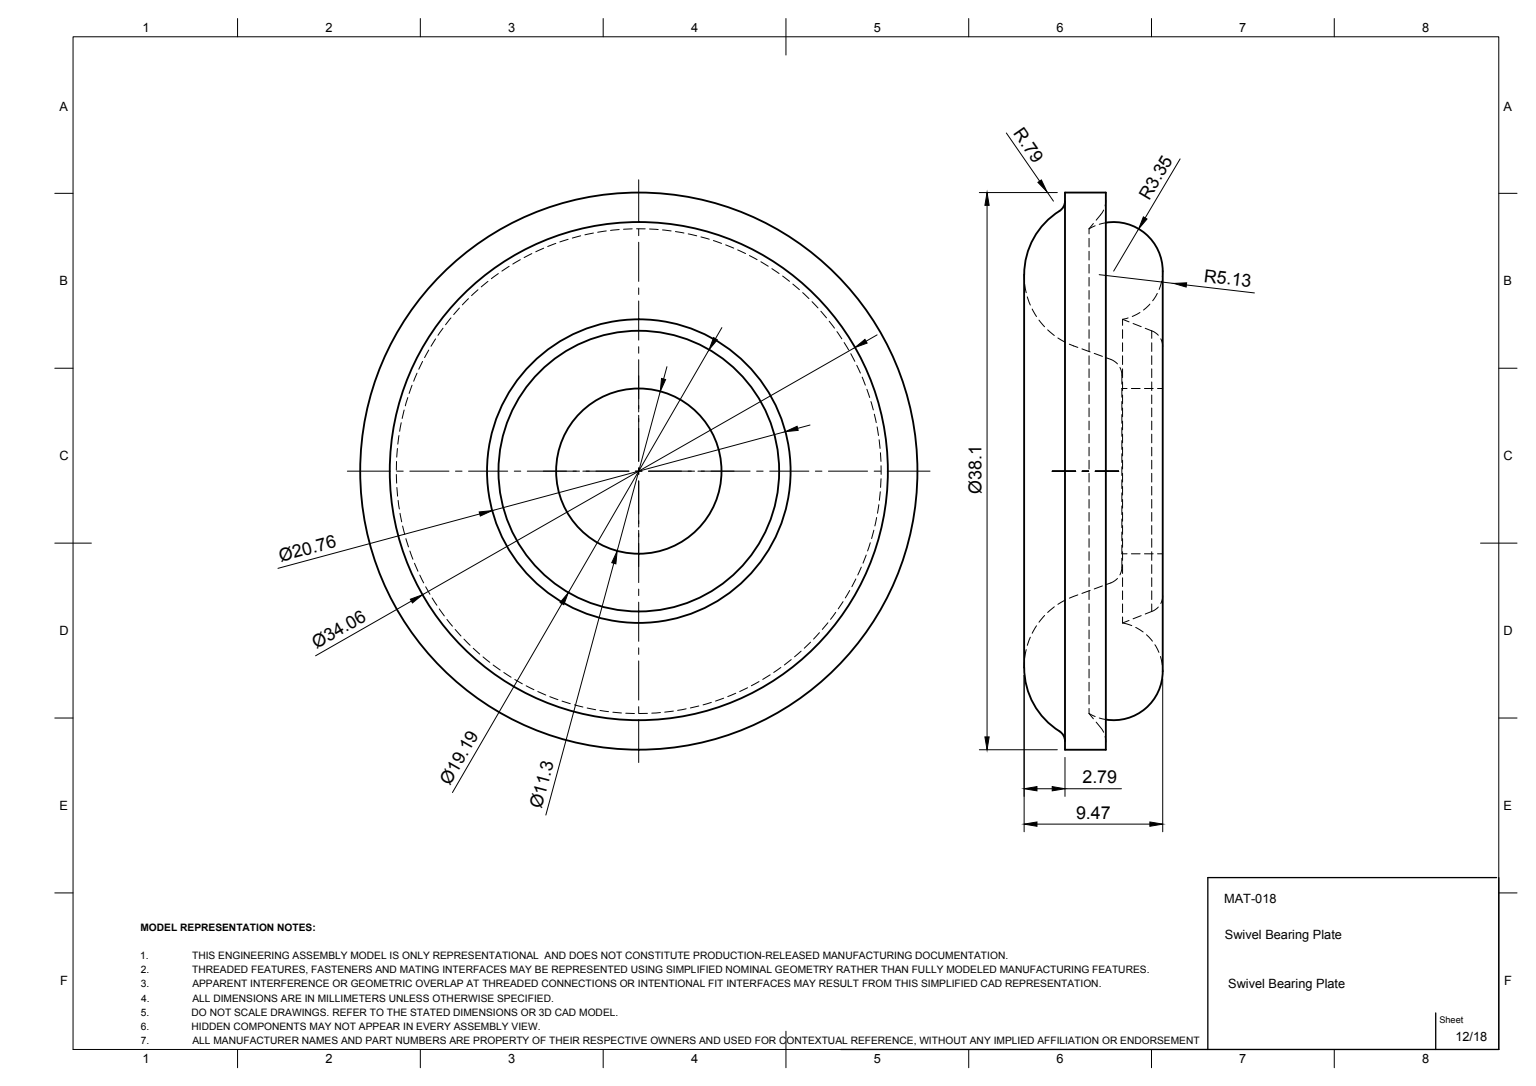
ISO-10303-21;
HEADER;
/* Generated by software containing ST-Developer
 * from STEP Tools, Inc. (www.steptools.com) 
 */

FILE_DESCRIPTION(
/* description */ ('STEP AP214'),
/* implementation_level */ '2;1');

FILE_NAME(
/* name */ 'Swivel Bearing Plate.step',
/* time_stamp */ '2026-11-14T06:16:09-08:00',
/* author */ (''),
/* organization */ (''),
/* preprocessor_version */ 'ST-DEVELOPER v20.2',
/* originating_system */ 'Autodesk Translation Framework v15.17.0.0',
/* authorisation */ '');

FILE_SCHEMA (('AUTOMOTIVE_DESIGN { 1 0 10303 214 3 1 1 }'));
ENDSEC;

DATA;
#10=MECHANICAL_DESIGN_GEOMETRIC_PRESENTATION_REPRESENTATION('',(#355),#18006);
#126=CONICAL_SURFACE('',#10555,9.59611131114252,0.375229267578829);
#127=CONICAL_SURFACE('',#10558,15.3208607241417,0.87573749484567);
#128=CONICAL_SURFACE('',#10579,8.56864389726312,0.349065850398865);
#241=TOROIDAL_SURFACE('',#10550,8.52204264558423,1.143);
#242=TOROIDAL_SURFACE('',#10561,18.5282252464232,1.5748);
#243=TOROIDAL_SURFACE('',#10567,18.4629769854638,0.7874);
#244=TOROIDAL_SURFACE('',#10571,13.4366,5.1308);
#245=TOROIDAL_SURFACE('',#10574,13.3900187959915,5.1308);
#246=TOROIDAL_SURFACE('',#10582,6.5656627838263,1.143);
#247=TOROIDAL_SURFACE('',#10585,13.6779,3.3528);
#323=SHAPE_REPRESENTATION_RELATIONSHIP('SRR','None',#18081,#339);
#339=ADVANCED_BREP_SHAPE_REPRESENTATION('',(#371),#17998);
#355=STYLED_ITEM('',(#18172),#371);
#371=MANIFOLD_SOLID_BREP('Body1',#9564);
#471=FACE_BOUND('',#1968,.T.);
#472=FACE_BOUND('',#1970,.T.);
#473=FACE_BOUND('',#1972,.T.);
#474=FACE_BOUND('',#1974,.T.);
#475=FACE_BOUND('',#1976,.T.);
#786=PLANE('',#10587);
#787=PLANE('',#10588);
#788=PLANE('',#10589);
#789=PLANE('',#10590);
#790=PLANE('',#10591);
#1287=FACE_OUTER_BOUND('',#1955,.T.);
#1288=FACE_OUTER_BOUND('',#1956,.T.);
#1289=FACE_OUTER_BOUND('',#1957,.T.);
#1290=FACE_OUTER_BOUND('',#1958,.T.);
#1291=FACE_OUTER_BOUND('',#1959,.T.);
#1292=FACE_OUTER_BOUND('',#1960,.T.);
#1293=FACE_OUTER_BOUND('',#1961,.T.);
#1294=FACE_OUTER_BOUND('',#1962,.T.);
#1295=FACE_OUTER_BOUND('',#1963,.T.);
#1296=FACE_OUTER_BOUND('',#1964,.T.);
#1297=FACE_OUTER_BOUND('',#1965,.T.);
#1298=FACE_OUTER_BOUND('',#1966,.T.);
#1299=FACE_OUTER_BOUND('',#1967,.T.);
#1300=FACE_OUTER_BOUND('',#1969,.T.);
#1301=FACE_OUTER_BOUND('',#1971,.T.);
#1302=FACE_OUTER_BOUND('',#1973,.T.);
#1303=FACE_OUTER_BOUND('',#1975,.T.);
#1955=EDGE_LOOP('',(#8296,#8297,#8298,#8299));
#1956=EDGE_LOOP('',(#8300,#8301,#8302,#8303,#8304));
#1957=EDGE_LOOP('',(#8305,#8306,#8307,#8308,#8309,#8310));
#1958=EDGE_LOOP('',(#8311,#8312,#8313,#8314));
#1959=EDGE_LOOP('',(#8315,#8316,#8317,#8318));
#1960=EDGE_LOOP('',(#8319,#8320,#8321,#8322));
#1961=EDGE_LOOP('',(#8323,#8324,#8325,#8326));
#1962=EDGE_LOOP('',(#8327,#8328,#8329,#8330));
#1963=EDGE_LOOP('',(#8331,#8332,#8333,#8334,#8335));
#1964=EDGE_LOOP('',(#8336,#8337,#8338,#8339,#8340,#8341));
#1965=EDGE_LOOP('',(#8342,#8343,#8344,#8345,#8346));
#1966=EDGE_LOOP('',(#8347,#8348,#8349,#8350,#8351));
#1967=EDGE_LOOP('',(#8352));
#1968=EDGE_LOOP('',(#8353));
#1969=EDGE_LOOP('',(#8354));
#1970=EDGE_LOOP('',(#8355));
#1971=EDGE_LOOP('',(#8356));
#1972=EDGE_LOOP('',(#8357));
#1973=EDGE_LOOP('',(#8358));
#1974=EDGE_LOOP('',(#8359));
#1975=EDGE_LOOP('',(#8360));
#1976=EDGE_LOOP('',(#8361));
#2752=LINE('',#17374,#3476);
#2753=LINE('',#17389,#3477);
#2754=LINE('',#17394,#3478);
#2755=LINE('',#17404,#3479);
#2756=LINE('',#17428,#3480);
#3476=VECTOR('',#13097,5.6515);
#3477=VECTOR('',#13116,9.59611131114252);
#3478=VECTOR('',#13121,15.3208607241417);
#3479=VECTOR('',#13134,19.05);
#3480=VECTOR('',#13165,8.56864389726312);
#3857=CIRCLE('',#10548,5.6515);
#3858=CIRCLE('',#10549,5.6515);
#3859=CIRCLE('',#10551,8.52204264558423);
#3860=CIRCLE('',#10552,1.143);
#3861=CIRCLE('',#10553,9.59611131114252);
#3862=CIRCLE('',#10554,9.59611131114252);
#3863=CIRCLE('',#10556,10.3807974512434);
#3864=CIRCLE('',#10557,10.3807974512434);
#3865=CIRCLE('',#10559,16.5763055377746);
#3866=CIRCLE('',#10560,17.5196750989302);
#3867=CIRCLE('',#10562,1.5748);
#3868=CIRCLE('',#10563,18.5282252464232);
#3869=CIRCLE('',#10565,19.05);
#3870=CIRCLE('',#10566,19.05);
#3871=CIRCLE('',#10568,18.4629769854638);
#3872=CIRCLE('',#10569,0.7874);
#3873=CIRCLE('',#10570,17.7942315496296);
#3874=CIRCLE('',#10572,5.1308);
#3875=CIRCLE('',#10573,13.4366);
#3876=CIRCLE('',#10575,13.3900187959915);
#3877=CIRCLE('',#10576,5.1308);
#3878=CIRCLE('',#10577,8.56864389726312);
#3879=CIRCLE('',#10578,8.56864389726312);
#3880=CIRCLE('',#10580,7.6397314493846);
#3881=CIRCLE('',#10581,7.6397314493846);
#3882=CIRCLE('',#10583,1.143);
#3883=CIRCLE('',#10584,6.5656627838263);
#3884=CIRCLE('',#10586,3.3528);
#4665=VERTEX_POINT('',#17371);
#4666=VERTEX_POINT('',#17373);
#4667=VERTEX_POINT('',#17377);
#4668=VERTEX_POINT('',#17379);
#4669=VERTEX_POINT('',#17381);
#4670=VERTEX_POINT('',#17385);
#4671=VERTEX_POINT('',#17386);
#4672=VERTEX_POINT('',#17391);
#4673=VERTEX_POINT('',#17393);
#4674=VERTEX_POINT('',#17397);
#4675=VERTEX_POINT('',#17401);
#4676=VERTEX_POINT('',#17403);
#4677=VERTEX_POINT('',#17407);
#4678=VERTEX_POINT('',#17409);
#4679=VERTEX_POINT('',#17413);
#4680=VERTEX_POINT('',#17417);
#4681=VERTEX_POINT('',#17419);
#4682=VERTEX_POINT('',#17421);
#4683=VERTEX_POINT('',#17425);
#4684=VERTEX_POINT('',#17426);
#4685=VERTEX_POINT('',#17431);
#5896=EDGE_CURVE('',#4665,#4665,#3857,.T.);
#5897=EDGE_CURVE('',#4665,#4666,#2752,.T.);
#5898=EDGE_CURVE('',#4666,#4666,#3858,.T.);
#5899=EDGE_CURVE('',#4667,#4667,#3859,.T.);
#5900=EDGE_CURVE('',#4667,#4668,#3860,.T.);
#5901=EDGE_CURVE('',#4668,#4669,#3861,.T.);
#5902=EDGE_CURVE('',#4669,#4668,#3862,.T.);
#5903=EDGE_CURVE('',#4670,#4671,#3863,.T.);
#5904=EDGE_CURVE('',#4671,#4670,#3864,.T.);
#5905=EDGE_CURVE('',#4671,#4669,#2753,.T.);
#5906=EDGE_CURVE('',#4672,#4672,#3865,.T.);
#5907=EDGE_CURVE('',#4672,#4673,#2754,.T.);
#5908=EDGE_CURVE('',#4673,#4673,#3866,.T.);
#5909=EDGE_CURVE('',#4673,#4674,#3867,.T.);
#5910=EDGE_CURVE('',#4674,#4674,#3868,.T.);
#5911=EDGE_CURVE('',#4675,#4675,#3869,.T.);
#5912=EDGE_CURVE('',#4675,#4676,#2755,.T.);
#5913=EDGE_CURVE('',#4676,#4676,#3870,.T.);
#5914=EDGE_CURVE('',#4677,#4677,#3871,.T.);
#5915=EDGE_CURVE('',#4677,#4678,#3872,.T.);
#5916=EDGE_CURVE('',#4678,#4678,#3873,.T.);
#5917=EDGE_CURVE('',#4678,#4679,#3874,.T.);
#5918=EDGE_CURVE('',#4679,#4679,#3875,.T.);
#5919=EDGE_CURVE('',#4680,#4680,#3876,.T.);
#5920=EDGE_CURVE('',#4680,#4681,#3877,.T.);
#5921=EDGE_CURVE('',#4681,#4682,#3878,.T.);
#5922=EDGE_CURVE('',#4682,#4681,#3879,.T.);
#5923=EDGE_CURVE('',#4683,#4684,#3880,.T.);
#5924=EDGE_CURVE('',#4684,#4682,#2756,.T.);
#5925=EDGE_CURVE('',#4684,#4683,#3881,.T.);
#5926=EDGE_CURVE('',#4683,#4685,#3882,.T.);
#5927=EDGE_CURVE('',#4685,#4685,#3883,.T.);
#5928=EDGE_CURVE('',#4670,#4672,#3884,.T.);
#8296=ORIENTED_EDGE('',*,*,#5896,.F.);
#8297=ORIENTED_EDGE('',*,*,#5897,.T.);
#8298=ORIENTED_EDGE('',*,*,#5898,.T.);
#8299=ORIENTED_EDGE('',*,*,#5897,.F.);
#8300=ORIENTED_EDGE('',*,*,#5899,.F.);
#8301=ORIENTED_EDGE('',*,*,#5900,.T.);
#8302=ORIENTED_EDGE('',*,*,#5901,.T.);
#8303=ORIENTED_EDGE('',*,*,#5902,.T.);
#8304=ORIENTED_EDGE('',*,*,#5900,.F.);
#8305=ORIENTED_EDGE('',*,*,#5903,.F.);
#8306=ORIENTED_EDGE('',*,*,#5904,.F.);
#8307=ORIENTED_EDGE('',*,*,#5905,.T.);
#8308=ORIENTED_EDGE('',*,*,#5901,.F.);
#8309=ORIENTED_EDGE('',*,*,#5902,.F.);
#8310=ORIENTED_EDGE('',*,*,#5905,.F.);
#8311=ORIENTED_EDGE('',*,*,#5906,.F.);
#8312=ORIENTED_EDGE('',*,*,#5907,.T.);
#8313=ORIENTED_EDGE('',*,*,#5908,.T.);
#8314=ORIENTED_EDGE('',*,*,#5907,.F.);
#8315=ORIENTED_EDGE('',*,*,#5908,.F.);
#8316=ORIENTED_EDGE('',*,*,#5909,.T.);
#8317=ORIENTED_EDGE('',*,*,#5910,.T.);
#8318=ORIENTED_EDGE('',*,*,#5909,.F.);
#8319=ORIENTED_EDGE('',*,*,#5911,.F.);
#8320=ORIENTED_EDGE('',*,*,#5912,.T.);
#8321=ORIENTED_EDGE('',*,*,#5913,.T.);
#8322=ORIENTED_EDGE('',*,*,#5912,.F.);
#8323=ORIENTED_EDGE('',*,*,#5914,.F.);
#8324=ORIENTED_EDGE('',*,*,#5915,.T.);
#8325=ORIENTED_EDGE('',*,*,#5916,.T.);
#8326=ORIENTED_EDGE('',*,*,#5915,.F.);
#8327=ORIENTED_EDGE('',*,*,#5916,.F.);
#8328=ORIENTED_EDGE('',*,*,#5917,.T.);
#8329=ORIENTED_EDGE('',*,*,#5918,.T.);
#8330=ORIENTED_EDGE('',*,*,#5917,.F.);
#8331=ORIENTED_EDGE('',*,*,#5919,.F.);
#8332=ORIENTED_EDGE('',*,*,#5920,.T.);
#8333=ORIENTED_EDGE('',*,*,#5921,.T.);
#8334=ORIENTED_EDGE('',*,*,#5922,.T.);
#8335=ORIENTED_EDGE('',*,*,#5920,.F.);
#8336=ORIENTED_EDGE('',*,*,#5923,.T.);
#8337=ORIENTED_EDGE('',*,*,#5924,.T.);
#8338=ORIENTED_EDGE('',*,*,#5921,.F.);
#8339=ORIENTED_EDGE('',*,*,#5922,.F.);
#8340=ORIENTED_EDGE('',*,*,#5924,.F.);
#8341=ORIENTED_EDGE('',*,*,#5925,.T.);
#8342=ORIENTED_EDGE('',*,*,#5923,.F.);
#8343=ORIENTED_EDGE('',*,*,#5926,.T.);
#8344=ORIENTED_EDGE('',*,*,#5927,.T.);
#8345=ORIENTED_EDGE('',*,*,#5926,.F.);
#8346=ORIENTED_EDGE('',*,*,#5925,.F.);
#8347=ORIENTED_EDGE('',*,*,#5903,.T.);
#8348=ORIENTED_EDGE('',*,*,#5904,.T.);
#8349=ORIENTED_EDGE('',*,*,#5928,.T.);
#8350=ORIENTED_EDGE('',*,*,#5906,.T.);
#8351=ORIENTED_EDGE('',*,*,#5928,.F.);
#8352=ORIENTED_EDGE('',*,*,#5918,.F.);
#8353=ORIENTED_EDGE('',*,*,#5919,.T.);
#8354=ORIENTED_EDGE('',*,*,#5913,.F.);
#8355=ORIENTED_EDGE('',*,*,#5914,.T.);
#8356=ORIENTED_EDGE('',*,*,#5911,.T.);
#8357=ORIENTED_EDGE('',*,*,#5910,.F.);
#8358=ORIENTED_EDGE('',*,*,#5899,.T.);
#8359=ORIENTED_EDGE('',*,*,#5898,.F.);
#8360=ORIENTED_EDGE('',*,*,#5927,.F.);
#8361=ORIENTED_EDGE('',*,*,#5896,.T.);
#8959=CYLINDRICAL_SURFACE('',#10547,5.6515);
#8960=CYLINDRICAL_SURFACE('',#10564,19.05);
#9426=ADVANCED_FACE('',(#1287),#8959,.F.);
#9427=ADVANCED_FACE('',(#1288),#241,.T.);
#9428=ADVANCED_FACE('',(#1289),#126,.T.);
#9429=ADVANCED_FACE('',(#1290),#127,.F.);
#9430=ADVANCED_FACE('',(#1291),#242,.T.);
#9431=ADVANCED_FACE('',(#1292),#8960,.T.);
#9432=ADVANCED_FACE('',(#1293),#243,.F.);
#9433=ADVANCED_FACE('',(#1294),#244,.T.);
#9434=ADVANCED_FACE('',(#1295),#245,.T.);
#9435=ADVANCED_FACE('',(#1296),#128,.F.);
#9436=ADVANCED_FACE('',(#1297),#246,.F.);
#9437=ADVANCED_FACE('',(#1298),#247,.T.);
#9438=ADVANCED_FACE('',(#1299,#471),#786,.T.);
#9439=ADVANCED_FACE('',(#1300,#472),#787,.T.);
#9440=ADVANCED_FACE('',(#1301,#473),#788,.T.);
#9441=ADVANCED_FACE('',(#1302,#474),#789,.T.);
#9442=ADVANCED_FACE('',(#1303,#475),#790,.T.);
#9564=CLOSED_SHELL('',(#9426,#9427,#9428,#9429,#9430,#9431,#9432,#9433,
#9434,#9435,#9436,#9437,#9438,#9439,#9440,#9441,#9442));
#10546=AXIS2_PLACEMENT_3D('',#17369,#13091,#13092);
#10547=AXIS2_PLACEMENT_3D('',#17370,#13093,#13094);
#10548=AXIS2_PLACEMENT_3D('',#17372,#13095,#13096);
#10549=AXIS2_PLACEMENT_3D('',#17375,#13098,#13099);
#10550=AXIS2_PLACEMENT_3D('',#17376,#13100,#13101);
#10551=AXIS2_PLACEMENT_3D('',#17378,#13102,#13103);
#10552=AXIS2_PLACEMENT_3D('',#17380,#13104,#13105);
#10553=AXIS2_PLACEMENT_3D('',#17382,#13106,#13107);
#10554=AXIS2_PLACEMENT_3D('',#17383,#13108,#13109);
#10555=AXIS2_PLACEMENT_3D('',#17384,#13110,#13111);
#10556=AXIS2_PLACEMENT_3D('',#17387,#13112,#13113);
#10557=AXIS2_PLACEMENT_3D('',#17388,#13114,#13115);
#10558=AXIS2_PLACEMENT_3D('',#17390,#13117,#13118);
#10559=AXIS2_PLACEMENT_3D('',#17392,#13119,#13120);
#10560=AXIS2_PLACEMENT_3D('',#17395,#13122,#13123);
#10561=AXIS2_PLACEMENT_3D('',#17396,#13124,#13125);
#10562=AXIS2_PLACEMENT_3D('',#17398,#13126,#13127);
#10563=AXIS2_PLACEMENT_3D('',#17399,#13128,#13129);
#10564=AXIS2_PLACEMENT_3D('',#17400,#13130,#13131);
#10565=AXIS2_PLACEMENT_3D('',#17402,#13132,#13133);
#10566=AXIS2_PLACEMENT_3D('',#17405,#13135,#13136);
#10567=AXIS2_PLACEMENT_3D('',#17406,#13137,#13138);
#10568=AXIS2_PLACEMENT_3D('',#17408,#13139,#13140);
#10569=AXIS2_PLACEMENT_3D('',#17410,#13141,#13142);
#10570=AXIS2_PLACEMENT_3D('',#17411,#13143,#13144);
#10571=AXIS2_PLACEMENT_3D('',#17412,#13145,#13146);
#10572=AXIS2_PLACEMENT_3D('',#17414,#13147,#13148);
#10573=AXIS2_PLACEMENT_3D('',#17415,#13149,#13150);
#10574=AXIS2_PLACEMENT_3D('',#17416,#13151,#13152);
#10575=AXIS2_PLACEMENT_3D('',#17418,#13153,#13154);
#10576=AXIS2_PLACEMENT_3D('',#17420,#13155,#13156);
#10577=AXIS2_PLACEMENT_3D('',#17422,#13157,#13158);
#10578=AXIS2_PLACEMENT_3D('',#17423,#13159,#13160);
#10579=AXIS2_PLACEMENT_3D('',#17424,#13161,#13162);
#10580=AXIS2_PLACEMENT_3D('',#17427,#13163,#13164);
#10581=AXIS2_PLACEMENT_3D('',#17429,#13166,#13167);
#10582=AXIS2_PLACEMENT_3D('',#17430,#13168,#13169);
#10583=AXIS2_PLACEMENT_3D('',#17432,#13170,#13171);
#10584=AXIS2_PLACEMENT_3D('',#17433,#13172,#13173);
#10585=AXIS2_PLACEMENT_3D('',#17434,#13174,#13175);
#10586=AXIS2_PLACEMENT_3D('',#17435,#13176,#13177);
#10587=AXIS2_PLACEMENT_3D('',#17436,#13178,#13179);
#10588=AXIS2_PLACEMENT_3D('',#17437,#13180,#13181);
#10589=AXIS2_PLACEMENT_3D('',#17438,#13182,#13183);
#10590=AXIS2_PLACEMENT_3D('',#17439,#13184,#13185);
#10591=AXIS2_PLACEMENT_3D('',#17440,#13186,#13187);
#13091=DIRECTION('axis',(0.,0.,1.));
#13092=DIRECTION('refdir',(1.,0.,0.));
#13093=DIRECTION('center_axis',(0.,-1.,0.));
#13094=DIRECTION('ref_axis',(0.,0.,-1.));
#13095=DIRECTION('center_axis',(0.,-1.,0.));
#13096=DIRECTION('ref_axis',(0.,0.,-1.));
#13097=DIRECTION('',(0.,-1.,0.));
#13098=DIRECTION('center_axis',(0.,-1.,0.));
#13099=DIRECTION('ref_axis',(0.,0.,-1.));
#13100=DIRECTION('center_axis',(0.,-1.,0.));
#13101=DIRECTION('ref_axis',(0.,0.,-1.));
#13102=DIRECTION('center_axis',(0.,-1.,0.));
#13103=DIRECTION('ref_axis',(0.,0.,-1.));
#13104=DIRECTION('center_axis',(-1.,0.,-1.22464679914735E-16));
#13105=DIRECTION('ref_axis',(-1.22464679914735E-16,0.,1.));
#13106=DIRECTION('center_axis',(0.,-1.,0.));
#13107=DIRECTION('ref_axis',(0.,0.,-1.));
#13108=DIRECTION('center_axis',(0.,-1.,0.));
#13109=DIRECTION('ref_axis',(0.,0.,-1.));
#13110=DIRECTION('center_axis',(0.,1.,0.));
#13111=DIRECTION('ref_axis',(0.,0.,1.));
#13112=DIRECTION('center_axis',(0.,1.,0.));
#13113=DIRECTION('ref_axis',(0.,0.,1.));
#13114=DIRECTION('center_axis',(0.,1.,0.));
#13115=DIRECTION('ref_axis',(0.,0.,1.));
#13116=DIRECTION('',(4.48815728875744E-17,-0.930423623041689,0.366485854687431));
#13117=DIRECTION('center_axis',(0.,-1.,0.));
#13118=DIRECTION('ref_axis',(0.,0.,-1.));
#13119=DIRECTION('center_axis',(0.,-1.,0.));
#13120=DIRECTION('ref_axis',(0.,0.,1.));
#13121=DIRECTION('',(-9.40548367125564E-17,-0.640430624519258,0.768016025339233));
#13122=DIRECTION('center_axis',(0.,-1.,0.));
#13123=DIRECTION('ref_axis',(0.,0.,-1.));
#13124=DIRECTION('center_axis',(0.,-1.,0.));
#13125=DIRECTION('ref_axis',(0.,0.,-1.));
#13126=DIRECTION('center_axis',(-1.,0.,-1.22464679914735E-16));
#13127=DIRECTION('ref_axis',(-1.22464679914735E-16,0.,1.));
#13128=DIRECTION('center_axis',(0.,-1.,0.));
#13129=DIRECTION('ref_axis',(0.,0.,-1.));
#13130=DIRECTION('center_axis',(0.,-1.,0.));
#13131=DIRECTION('ref_axis',(0.,0.,-1.));
#13132=DIRECTION('center_axis',(0.,-1.,0.));
#13133=DIRECTION('ref_axis',(0.,0.,-1.));
#13134=DIRECTION('',(0.,1.,0.));
#13135=DIRECTION('center_axis',(0.,-1.,0.));
#13136=DIRECTION('ref_axis',(0.,0.,-1.));
#13137=DIRECTION('center_axis',(0.,-1.,0.));
#13138=DIRECTION('ref_axis',(0.,0.,-1.));
#13139=DIRECTION('center_axis',(0.,-1.,0.));
#13140=DIRECTION('ref_axis',(0.,0.,-1.));
#13141=DIRECTION('center_axis',(1.,0.,1.22464679914735E-16));
#13142=DIRECTION('ref_axis',(-1.22464679914735E-16,0.,1.));
#13143=DIRECTION('center_axis',(0.,-1.,0.));
#13144=DIRECTION('ref_axis',(0.,0.,-1.));
#13145=DIRECTION('center_axis',(0.,-1.,0.));
#13146=DIRECTION('ref_axis',(0.,0.,-1.));
#13147=DIRECTION('center_axis',(-1.,0.,-1.22464679914735E-16));
#13148=DIRECTION('ref_axis',(-1.22464679914735E-16,0.,1.));
#13149=DIRECTION('center_axis',(0.,-1.,0.));
#13150=DIRECTION('ref_axis',(0.,0.,-1.));
#13151=DIRECTION('center_axis',(0.,-1.,0.));
#13152=DIRECTION('ref_axis',(0.,0.,-1.));
#13153=DIRECTION('center_axis',(0.,-1.,0.));
#13154=DIRECTION('ref_axis',(0.,0.,-1.));
#13155=DIRECTION('center_axis',(-1.,0.,-1.22464679914735E-16));
#13156=DIRECTION('ref_axis',(-1.22464679914735E-16,0.,1.));
#13157=DIRECTION('center_axis',(0.,-1.,0.));
#13158=DIRECTION('ref_axis',(0.,0.,-1.));
#13159=DIRECTION('center_axis',(0.,-1.,0.));
#13160=DIRECTION('ref_axis',(0.,0.,-1.));
#13161=DIRECTION('center_axis',(0.,1.,0.));
#13162=DIRECTION('ref_axis',(0.,0.,1.));
#13163=DIRECTION('center_axis',(0.,-1.,0.));
#13164=DIRECTION('ref_axis',(0.,0.,-1.));
#13165=DIRECTION('',(-4.18853873767698E-17,0.939692620785909,-0.342020143325668));
#13166=DIRECTION('center_axis',(0.,-1.,0.));
#13167=DIRECTION('ref_axis',(0.,0.,-1.));
#13168=DIRECTION('center_axis',(0.,-1.,0.));
#13169=DIRECTION('ref_axis',(0.,0.,-1.));
#13170=DIRECTION('center_axis',(1.,0.,1.22464679914735E-16));
#13171=DIRECTION('ref_axis',(-1.22464679914735E-16,0.,1.));
#13172=DIRECTION('center_axis',(0.,-1.,0.));
#13173=DIRECTION('ref_axis',(0.,0.,-1.));
#13174=DIRECTION('center_axis',(0.,-1.,0.));
#13175=DIRECTION('ref_axis',(0.,0.,-1.));
#13176=DIRECTION('center_axis',(-1.,0.,-1.22464679914735E-16));
#13177=DIRECTION('ref_axis',(-1.22464679914735E-16,0.,1.));
#13178=DIRECTION('center_axis',(0.,1.,0.));
#13179=DIRECTION('ref_axis',(1.,0.,0.));
#13180=DIRECTION('center_axis',(0.,1.,0.));
#13181=DIRECTION('ref_axis',(1.,0.,0.));
#13182=DIRECTION('center_axis',(0.,-1.,0.));
#13183=DIRECTION('ref_axis',(0.,0.,-1.));
#13184=DIRECTION('center_axis',(0.,-1.,0.));
#13185=DIRECTION('ref_axis',(0.,0.,-1.));
#13186=DIRECTION('center_axis',(0.,1.,0.));
#13187=DIRECTION('ref_axis',(1.,0.,0.));
#17369=CARTESIAN_POINT('',(0.,0.,0.));
#17370=CARTESIAN_POINT('Origin',(0.,-9.4742,0.));
#17371=CARTESIAN_POINT('',(-6.92109138538127E-16,-6.6802,5.6515));
#17372=CARTESIAN_POINT('Origin',(0.,-6.6802,0.));
#17373=CARTESIAN_POINT('',(-6.92109138538127E-16,-9.4742,5.6515));
#17374=CARTESIAN_POINT('',(-6.92109138538127E-16,-9.4742,5.6515));
#17375=CARTESIAN_POINT('Origin',(0.,-9.4742,0.));
#17376=CARTESIAN_POINT('Origin',(0.,-8.3312,0.));
#17377=CARTESIAN_POINT('',(-1.0436492248112E-15,-9.4742,8.52204264558423));
#17378=CARTESIAN_POINT('Origin',(0.,-9.4742,0.));
#17379=CARTESIAN_POINT('',(-1.17518470014524E-15,-8.72212902382124,9.59611131114252));
#17380=CARTESIAN_POINT('Origin',(-1.0436492248112E-15,-8.3312,8.52204264558423));
#17381=CARTESIAN_POINT('',(1.22323286863573E-15,-8.72212902382124,-9.59611131114252));
#17382=CARTESIAN_POINT('Origin',(0.,-8.72212902382124,0.));
#17383=CARTESIAN_POINT('Origin',(0.,-8.72212902382124,0.));
#17384=CARTESIAN_POINT('Origin',(0.,-8.72212902382124,0.));
#17385=CARTESIAN_POINT('',(1.65064649448932E-15,-6.72999068591485,10.3807974512434));
#17386=CARTESIAN_POINT('',(-1.27128103712622E-15,-6.72999068591485,-10.3807974512434));
#17387=CARTESIAN_POINT('Origin',(0.,-6.72999068591485,0.));
#17388=CARTESIAN_POINT('Origin',(0.,-6.72999068591485,0.));
#17389=CARTESIAN_POINT('',(-1.17518470014524E-15,-8.72212902382124,-9.59611131114252));
#17390=CARTESIAN_POINT('Origin',(0.,-3.38913168859475,0.));
#17391=CARTESIAN_POINT('',(-2.03001195185241E-15,-4.43601779450536,16.5763055377745));
#17392=CARTESIAN_POINT('Origin',(0.,-4.43601779450534,0.));
#17393=CARTESIAN_POINT('',(-2.14554140320065E-15,-5.22267163670422,17.5196750989302));
#17394=CARTESIAN_POINT('',(-1.87626430460025E-15,-3.38913168859475,15.3208607241417));
#17395=CARTESIAN_POINT('Origin',(0.,-5.22267163670421,0.));
#17396=CARTESIAN_POINT('Origin',(0.,-4.0132,0.));
#17397=CARTESIAN_POINT('',(-2.26905317419133E-15,-5.588,18.5282252464232));
#17398=CARTESIAN_POINT('Origin',(-2.26905317419134E-15,-4.0132,18.5282252464232));
#17399=CARTESIAN_POINT('Origin',(0.,-5.588,0.));
#17400=CARTESIAN_POINT('Origin',(0.,-9.4742,0.));
#17401=CARTESIAN_POINT('',(-2.33295215237571E-15,-5.588,19.05));
#17402=CARTESIAN_POINT('Origin',(0.,-5.588,0.));
#17403=CARTESIAN_POINT('',(-2.33295215237571E-15,-2.794,19.05));
#17404=CARTESIAN_POINT('',(-2.33295215237571E-15,-9.4742,19.05));
#17405=CARTESIAN_POINT('Origin',(0.,-2.794,0.));
#17406=CARTESIAN_POINT('Origin',(0.,-2.0066,0.));
#17407=CARTESIAN_POINT('',(-2.26106256679795E-15,-2.794,18.4629769854638));
#17408=CARTESIAN_POINT('Origin',(0.,-2.794,0.));
#17409=CARTESIAN_POINT('',(-2.17916487105407E-15,-2.4222660944206,17.7942315496296));
#17410=CARTESIAN_POINT('Origin',(-2.26106256679795E-15,-2.0066,18.4629769854638));
#17411=CARTESIAN_POINT('Origin',(0.,-2.4222660944206,0.));
#17412=CARTESIAN_POINT('Origin',(0.,-5.1308,0.));
#17413=CARTESIAN_POINT('',(-1.64550891814233E-15,0.,13.4366));
#17414=CARTESIAN_POINT('Origin',(-1.64550891814233E-15,-5.1308,13.4366));
#17415=CARTESIAN_POINT('Origin',(0.,0.,0.));
#17416=CARTESIAN_POINT('Origin',(0.,-5.1308,0.));
#17417=CARTESIAN_POINT('',(-1.63980436590338E-15,0.,13.3900187959915));
#17418=CARTESIAN_POINT('Origin',(0.,0.,0.));
#17419=CARTESIAN_POINT('',(-1.04935623218168E-15,-3.37596304862466,8.56864389726312));
#17420=CARTESIAN_POINT('Origin',(-1.63980436590338E-15,-5.1308,13.3900187959915));
#17421=CARTESIAN_POINT('',(1.04935623218168E-15,-3.37596304862466,-8.56864389726312));
#17422=CARTESIAN_POINT('Origin',(0.,-3.37596304862466,0.));
#17423=CARTESIAN_POINT('Origin',(0.,-3.37596304862466,0.));
#17424=CARTESIAN_POINT('Origin',(0.,-3.37596304862466,0.));
#17425=CARTESIAN_POINT('',(9.35597266583422E-16,-5.92812902382124,7.6397314493846));
#17426=CARTESIAN_POINT('',(-9.35597266583421E-16,-5.92812902382124,-7.63973144938459));
#17427=CARTESIAN_POINT('Origin',(0.,-5.92812902382124,0.));
#17428=CARTESIAN_POINT('',(-1.04935623218168E-15,-3.37596304862466,-8.56864389726312));
#17429=CARTESIAN_POINT('Origin',(0.,-5.92812902382124,0.));
#17430=CARTESIAN_POINT('Origin',(0.,-5.5372,0.));
#17431=CARTESIAN_POINT('',(-8.04061791249378E-16,-6.6802,6.5656627838263));
#17432=CARTESIAN_POINT('Origin',(-8.04061791249378E-16,-5.5372,6.5656627838263));
#17433=CARTESIAN_POINT('Origin',(0.,-6.6802,0.));
#17434=CARTESIAN_POINT('Origin',(0.,-6.1214,0.));
#17435=CARTESIAN_POINT('Origin',(-1.67505964540576E-15,-6.1214,13.6779));
#17436=CARTESIAN_POINT('Origin',(13.4366,0.,0.));
#17437=CARTESIAN_POINT('Origin',(19.05,-2.794,0.));
#17438=CARTESIAN_POINT('Origin',(18.5282252464232,-5.588,0.));
#17439=CARTESIAN_POINT('Origin',(5.6515,-9.4742,0.));
#17440=CARTESIAN_POINT('Origin',(6.5656627838263,-6.6802,0.));
#17978=UNCERTAINTY_MEASURE_WITH_UNIT(LENGTH_MEASURE(0.01),#18007,
'DISTANCE_ACCURACY_VALUE',
'Maximum model space distance between geometric entities at asserted c
onnectivities');
#17986=UNCERTAINTY_MEASURE_WITH_UNIT(LENGTH_MEASURE(0.01),#18007,
'DISTANCE_ACCURACY_VALUE',
'Maximum model space distance between geometric entities at asserted c
onnectivities');
#17998=(
GEOMETRIC_REPRESENTATION_CONTEXT(3)
GLOBAL_UNCERTAINTY_ASSIGNED_CONTEXT((#17978))
GLOBAL_UNIT_ASSIGNED_CONTEXT((#18007,#18009,#18010))
REPRESENTATION_CONTEXT('','3D')
);
#18006=(
GEOMETRIC_REPRESENTATION_CONTEXT(3)
GLOBAL_UNCERTAINTY_ASSIGNED_CONTEXT((#17986))
GLOBAL_UNIT_ASSIGNED_CONTEXT((#18007,#18009,#18010))
REPRESENTATION_CONTEXT('','3D')
);
#18007=(
LENGTH_UNIT()
NAMED_UNIT(*)
SI_UNIT(.MILLI.,.METRE.)
);
#18009=(
NAMED_UNIT(*)
PLANE_ANGLE_UNIT()
SI_UNIT($,.RADIAN.)
);
#18010=(
NAMED_UNIT(*)
SI_UNIT($,.STERADIAN.)
SOLID_ANGLE_UNIT()
);
#18022=SHAPE_DEFINITION_REPRESENTATION(#18041,#18081);
#18041=PRODUCT_DEFINITION_SHAPE('',$,#18101);
#18081=SHAPE_REPRESENTATION('',(#10546),#17998);
#18089=PRODUCT_DEFINITION_CONTEXT('part definition',#18148,'design');
#18101=PRODUCT_DEFINITION('Swivel Bearing Plate','Swivel Bearing Plate',
#18120,#18089);
#18120=PRODUCT_DEFINITION_FORMATION('',$,#18161);
#18148=APPLICATION_CONTEXT(
'Core Data for Automotive Mechanical Design Process');
#18149=PRODUCT_CONTEXT('part definition',#18148,'mechanical');
#18161=PRODUCT('Swivel Bearing Plate','Swivel Bearing Plate',$,(#18149));
#18172=PRESENTATION_STYLE_ASSIGNMENT((#18176));
#18176=SURFACE_STYLE_USAGE(.BOTH.,#18180);
#18180=SURFACE_SIDE_STYLE('',(#18184));
#18184=SURFACE_STYLE_FILL_AREA(#18188);
#18188=FILL_AREA_STYLE('Opaque(97,158,199)',(#18192));
#18192=FILL_AREA_STYLE_COLOUR('Opaque(97,158,199)',#18196);
#18196=COLOUR_RGB('Opaque(97,158,199)',0.380392156862745,0.619607843137255,
0.780392156862745);
ENDSEC;
END-ISO-10303-21;
